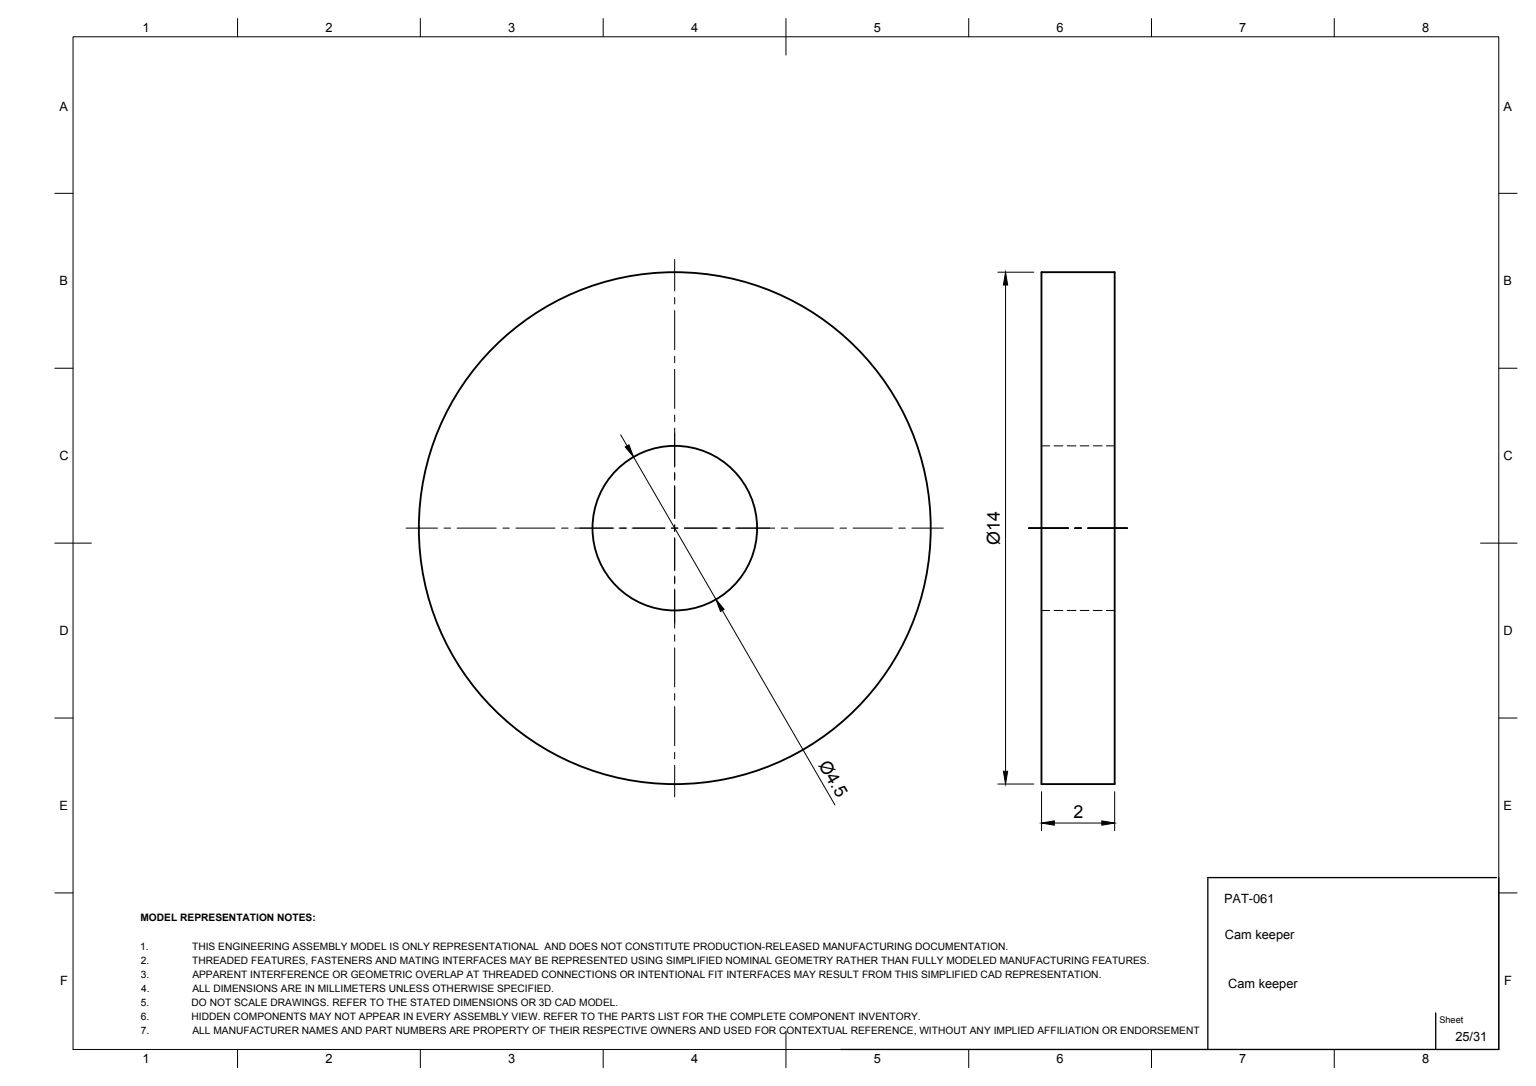
ISO-10303-21;
HEADER;
/* Generated by software containing ST-Developer
 * from STEP Tools, Inc. (www.steptools.com) 
 */

FILE_DESCRIPTION(
/* description */ ('Compact intermittent indexer'),
/* implementation_level */ '2;1');

FILE_NAME(
/* name */ 'Cam keeper.step',
/* time_stamp */ '2026-10-29T16:32:17-07:00',
/* author */ (''),
/* organization */ (''),
/* preprocessor_version */ 'ST-DEVELOPER v20.2',
/* originating_system */ 'Autodesk Translation Framework v15.17.0.0',
/* authorisation */ '');

FILE_SCHEMA (('AUTOMOTIVE_DESIGN { 1 0 10303 214 3 1 1 }'));
ENDSEC;

DATA;
#10=MECHANICAL_DESIGN_GEOMETRIC_PRESENTATION_REPRESENTATION('',(#282),#10837);
#226=SHAPE_REPRESENTATION_RELATIONSHIP('SRR','None',#10962,#250);
#250=ADVANCED_BREP_SHAPE_REPRESENTATION('',(#313),#10829);
#282=STYLED_ITEM('',(#11152),#313);
#313=MANIFOLD_SOLID_BREP('Body1',#5655);
#450=FACE_BOUND('',#1308,.T.);
#451=FACE_BOUND('',#1310,.T.);
#585=PLANE('',#6432);
#586=PLANE('',#6433);
#880=FACE_OUTER_BOUND('',#1305,.T.);
#881=FACE_OUTER_BOUND('',#1306,.T.);
#882=FACE_OUTER_BOUND('',#1307,.T.);
#883=FACE_OUTER_BOUND('',#1309,.T.);
#1305=EDGE_LOOP('',(#4648,#4649,#4650,#4651));
#1306=EDGE_LOOP('',(#4652,#4653,#4654,#4655));
#1307=EDGE_LOOP('',(#4656));
#1308=EDGE_LOOP('',(#4657));
#1309=EDGE_LOOP('',(#4658));
#1310=EDGE_LOOP('',(#4659));
#1629=LINE('',#10076,#1987);
#1630=LINE('',#10082,#1988);
#1987=VECTOR('',#7863,0.225);
#1988=VECTOR('',#7870,0.7);
#2391=CIRCLE('',#6427,0.225);
#2392=CIRCLE('',#6428,0.225);
#2393=CIRCLE('',#6430,0.7);
#2394=CIRCLE('',#6431,0.7);
#2803=VERTEX_POINT('',#10073);
#2804=VERTEX_POINT('',#10075);
#2805=VERTEX_POINT('',#10079);
#2806=VERTEX_POINT('',#10081);
#3446=EDGE_CURVE('',#2803,#2803,#2391,.T.);
#3447=EDGE_CURVE('',#2803,#2804,#1629,.T.);
#3448=EDGE_CURVE('',#2804,#2804,#2392,.T.);
#3449=EDGE_CURVE('',#2805,#2805,#2393,.T.);
#3450=EDGE_CURVE('',#2805,#2806,#1630,.T.);
#3451=EDGE_CURVE('',#2806,#2806,#2394,.T.);
#4648=ORIENTED_EDGE('',*,*,#3446,.F.);
#4649=ORIENTED_EDGE('',*,*,#3447,.T.);
#4650=ORIENTED_EDGE('',*,*,#3448,.T.);
#4651=ORIENTED_EDGE('',*,*,#3447,.F.);
#4652=ORIENTED_EDGE('',*,*,#3449,.F.);
#4653=ORIENTED_EDGE('',*,*,#3450,.T.);
#4654=ORIENTED_EDGE('',*,*,#3451,.T.);
#4655=ORIENTED_EDGE('',*,*,#3450,.F.);
#4656=ORIENTED_EDGE('',*,*,#3449,.T.);
#4657=ORIENTED_EDGE('',*,*,#3446,.T.);
#4658=ORIENTED_EDGE('',*,*,#3451,.F.);
#4659=ORIENTED_EDGE('',*,*,#3448,.F.);
#5260=CYLINDRICAL_SURFACE('',#6426,0.225);
#5261=CYLINDRICAL_SURFACE('',#6429,0.7);
#5523=ADVANCED_FACE('',(#880),#5260,.F.);
#5524=ADVANCED_FACE('',(#881),#5261,.T.);
#5525=ADVANCED_FACE('',(#882,#450),#585,.T.);
#5526=ADVANCED_FACE('',(#883,#451),#586,.F.);
#5655=CLOSED_SHELL('',(#5523,#5524,#5525,#5526));
#6425=AXIS2_PLACEMENT_3D('',#10071,#7857,#7858);
#6426=AXIS2_PLACEMENT_3D('',#10072,#7859,#7860);
#6427=AXIS2_PLACEMENT_3D('',#10074,#7861,#7862);
#6428=AXIS2_PLACEMENT_3D('',#10077,#7864,#7865);
#6429=AXIS2_PLACEMENT_3D('',#10078,#7866,#7867);
#6430=AXIS2_PLACEMENT_3D('',#10080,#7868,#7869);
#6431=AXIS2_PLACEMENT_3D('',#10083,#7871,#7872);
#6432=AXIS2_PLACEMENT_3D('',#10084,#7873,#7874);
#6433=AXIS2_PLACEMENT_3D('',#10085,#7875,#7876);
#7857=DIRECTION('axis',(0.,0.,1.));
#7858=DIRECTION('refdir',(1.,0.,0.));
#7859=DIRECTION('center_axis',(0.,0.,1.));
#7860=DIRECTION('ref_axis',(1.,0.,0.));
#7861=DIRECTION('center_axis',(0.,0.,-1.));
#7862=DIRECTION('ref_axis',(1.,0.,0.));
#7863=DIRECTION('',(0.,0.,-1.));
#7864=DIRECTION('center_axis',(0.,0.,-1.));
#7865=DIRECTION('ref_axis',(1.,0.,0.));
#7866=DIRECTION('center_axis',(0.,0.,1.));
#7867=DIRECTION('ref_axis',(1.,0.,0.));
#7868=DIRECTION('center_axis',(0.,0.,1.));
#7869=DIRECTION('ref_axis',(1.,0.,0.));
#7870=DIRECTION('',(0.,0.,-1.));
#7871=DIRECTION('center_axis',(0.,0.,1.));
#7872=DIRECTION('ref_axis',(1.,0.,0.));
#7873=DIRECTION('center_axis',(0.,0.,1.));
#7874=DIRECTION('ref_axis',(1.,0.,0.));
#7875=DIRECTION('center_axis',(0.,0.,1.));
#7876=DIRECTION('ref_axis',(1.,0.,0.));
#10071=CARTESIAN_POINT('',(0.,0.,0.));
#10072=CARTESIAN_POINT('Origin',(0.,0.,6.8));
#10073=CARTESIAN_POINT('',(-0.225,-2.75545529808154E-17,7.));
#10074=CARTESIAN_POINT('Origin',(0.,0.,7.));
#10075=CARTESIAN_POINT('',(-0.225,-2.75545529808154E-17,6.8));
#10076=CARTESIAN_POINT('',(-0.225,-2.75545529808154E-17,6.8));
#10077=CARTESIAN_POINT('Origin',(0.,0.,6.8));
#10078=CARTESIAN_POINT('Origin',(0.,0.,6.8));
#10079=CARTESIAN_POINT('',(-0.7,-8.57252759403147E-17,7.));
#10080=CARTESIAN_POINT('Origin',(0.,0.,7.));
#10081=CARTESIAN_POINT('',(-0.7,-8.57252759403147E-17,6.8));
#10082=CARTESIAN_POINT('',(-0.7,-8.57252759403147E-17,6.8));
#10083=CARTESIAN_POINT('Origin',(0.,0.,6.8));
#10084=CARTESIAN_POINT('Origin',(0.,0.,7.));
#10085=CARTESIAN_POINT('Origin',(0.,0.,6.8));
#10799=UNCERTAINTY_MEASURE_WITH_UNIT(LENGTH_MEASURE(0.001),#10838,
'DISTANCE_ACCURACY_VALUE',
'Maximum model space distance between geometric entities at asserted c
onnectivities');
#10807=UNCERTAINTY_MEASURE_WITH_UNIT(LENGTH_MEASURE(0.001),#10838,
'DISTANCE_ACCURACY_VALUE',
'Maximum model space distance between geometric entities at asserted c
onnectivities');
#10829=(
GEOMETRIC_REPRESENTATION_CONTEXT(3)
GLOBAL_UNCERTAINTY_ASSIGNED_CONTEXT((#10799))
GLOBAL_UNIT_ASSIGNED_CONTEXT((#10838,#10840,#10841))
REPRESENTATION_CONTEXT('','3D')
);
#10837=(
GEOMETRIC_REPRESENTATION_CONTEXT(3)
GLOBAL_UNCERTAINTY_ASSIGNED_CONTEXT((#10807))
GLOBAL_UNIT_ASSIGNED_CONTEXT((#10838,#10840,#10841))
REPRESENTATION_CONTEXT('','3D')
);
#10838=(
LENGTH_UNIT()
NAMED_UNIT(*)
SI_UNIT(.CENTI.,.METRE.)
);
#10840=(
NAMED_UNIT(*)
PLANE_ANGLE_UNIT()
SI_UNIT($,.RADIAN.)
);
#10841=(
NAMED_UNIT(*)
SI_UNIT($,.STERADIAN.)
SOLID_ANGLE_UNIT()
);
#10863=SHAPE_DEFINITION_REPRESENTATION(#10897,#10962);
#10897=PRODUCT_DEFINITION_SHAPE('',$,#10992);
#10962=SHAPE_REPRESENTATION('',(#6425),#10829);
#10970=PRODUCT_DEFINITION_CONTEXT('part definition',#11059,'design');
#10992=PRODUCT_DEFINITION('Cam keeper','Cam keeper',#11021,#10970);
#11021=PRODUCT_DEFINITION_FORMATION('',$,#11082);
#11059=APPLICATION_CONTEXT(
'Core Data for Automotive Mechanical Design Process');
#11060=PRODUCT_CONTEXT('part definition',#11059,'mechanical');
#11082=PRODUCT('Cam keeper','Cam keeper','Cam keeper',(#11060));
#11146=COLOUR_RGB('Light Blue',0.38,0.62,0.78);
#11147=FILL_AREA_STYLE_COLOUR('',#11146);
#11148=FILL_AREA_STYLE('',(#11147));
#11149=SURFACE_STYLE_FILL_AREA(#11148);
#11150=SURFACE_SIDE_STYLE('',(#11149));
#11151=SURFACE_STYLE_USAGE(.BOTH.,#11150);
#11152=PRESENTATION_STYLE_ASSIGNMENT((#11151));
ENDSEC;
END-ISO-10303-21;
